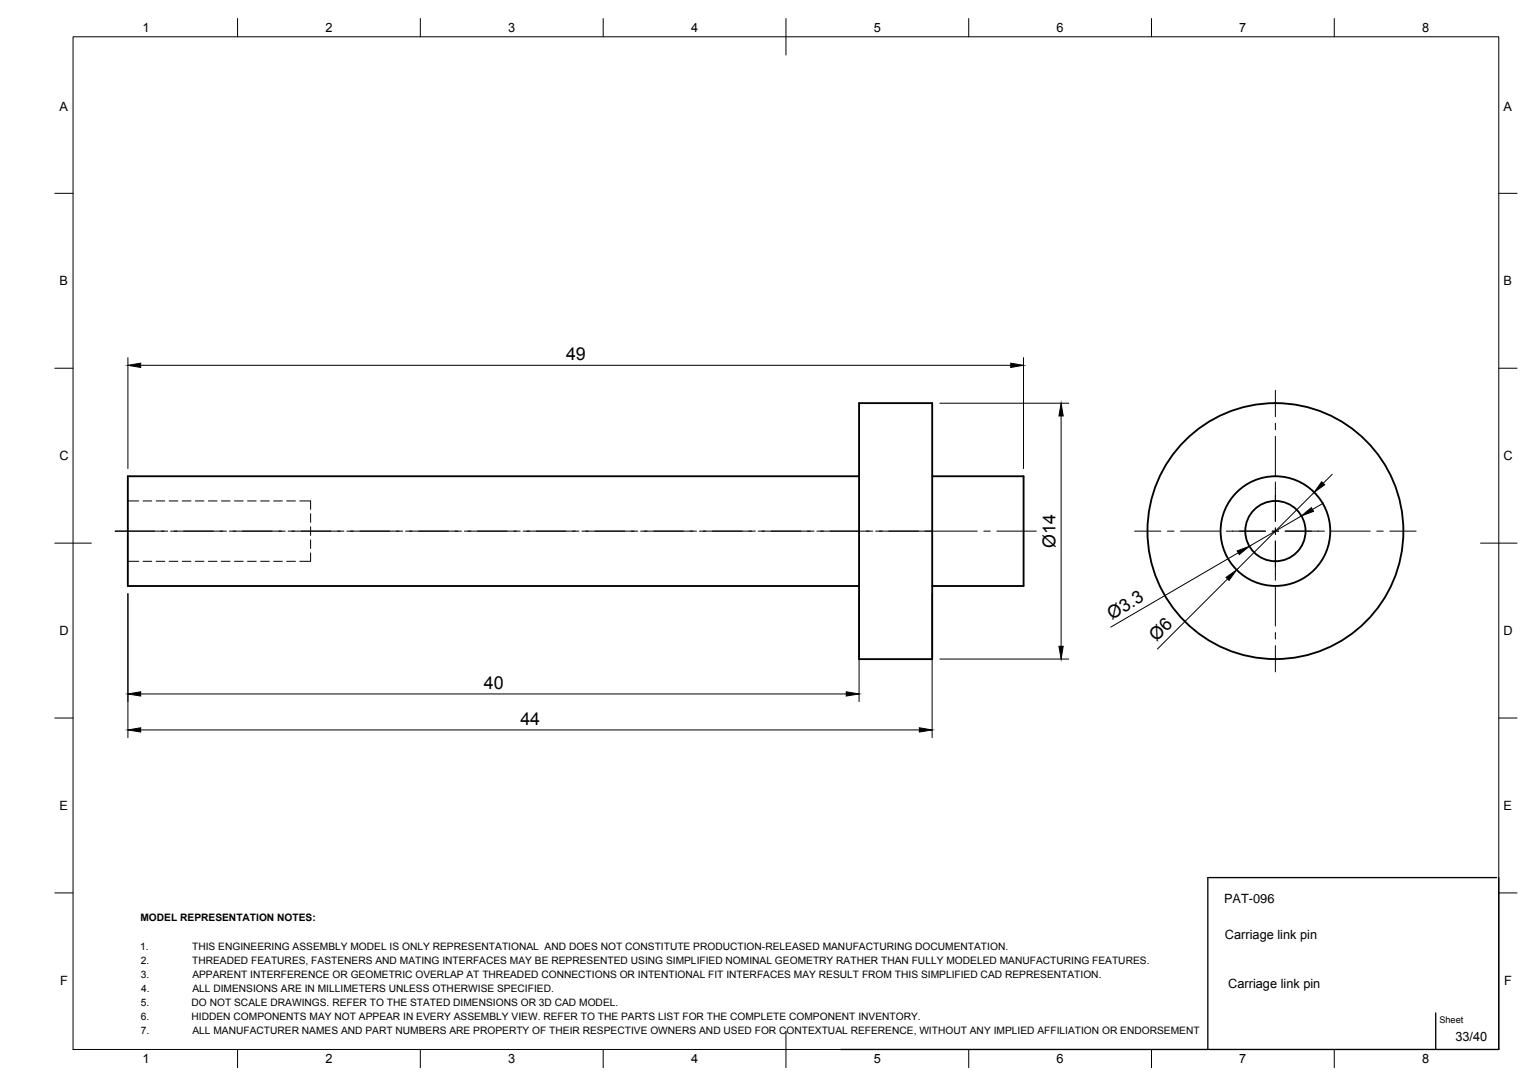
ISO-10303-21;
HEADER;
/* Generated by software containing ST-Developer
 * from STEP Tools, Inc. (www.steptools.com) 
 */

FILE_DESCRIPTION(
/* description */ ('PAT-096'),
/* implementation_level */ '2;1');

FILE_NAME(
/* name */ 'Carriage link pin.step',
/* time_stamp */ '2026-10-29T17:03:14-07:00',
/* author */ (''),
/* organization */ (''),
/* preprocessor_version */ 'ST-DEVELOPER v20.2',
/* originating_system */ 'Autodesk Translation Framework v15.17.0.0',
/* authorisation */ '');

FILE_SCHEMA (('AUTOMOTIVE_DESIGN { 1 0 10303 214 3 1 1 }'));
ENDSEC;

DATA;
#10=MECHANICAL_DESIGN_GEOMETRIC_PRESENTATION_REPRESENTATION('',(#428),#10650);
#358=SHAPE_REPRESENTATION_RELATIONSHIP('SRR','None',#10822,#389);
#389=ADVANCED_BREP_SHAPE_REPRESENTATION('',(#465),#10640);
#428=STYLED_ITEM('',(#11064),#465);
#465=MANIFOLD_SOLID_BREP('Body1',#5563);
#570=FACE_BOUND('',#1476,.T.);
#571=FACE_BOUND('',#1478,.T.);
#572=FACE_BOUND('',#1483,.T.);
#738=PLANE('',#6453);
#739=PLANE('',#6454);
#740=PLANE('',#6457);
#741=PLANE('',#6465);
#742=PLANE('',#6466);
#1040=FACE_OUTER_BOUND('',#1473,.T.);
#1041=FACE_OUTER_BOUND('',#1474,.T.);
#1042=FACE_OUTER_BOUND('',#1475,.T.);
#1043=FACE_OUTER_BOUND('',#1477,.T.);
#1044=FACE_OUTER_BOUND('',#1479,.T.);
#1045=FACE_OUTER_BOUND('',#1480,.T.);
#1046=FACE_OUTER_BOUND('',#1481,.T.);
#1047=FACE_OUTER_BOUND('',#1482,.T.);
#1048=FACE_OUTER_BOUND('',#1484,.T.);
#1473=EDGE_LOOP('',(#4743,#4744,#4745,#4746));
#1474=EDGE_LOOP('',(#4747));
#1475=EDGE_LOOP('',(#4748));
#1476=EDGE_LOOP('',(#4749));
#1477=EDGE_LOOP('',(#4750));
#1478=EDGE_LOOP('',(#4751));
#1479=EDGE_LOOP('',(#4752,#4753,#4754,#4755));
#1480=EDGE_LOOP('',(#4756,#4757,#4758,#4759));
#1481=EDGE_LOOP('',(#4760,#4761,#4762,#4763));
#1482=EDGE_LOOP('',(#4764));
#1483=EDGE_LOOP('',(#4765));
#1484=EDGE_LOOP('',(#4766));
#1836=LINE('',#10153,#2165);
#1837=LINE('',#10167,#2166);
#1838=LINE('',#10170,#2167);
#1839=LINE('',#10175,#2168);
#2165=VECTOR('',#7980,0.165);
#2166=VECTOR('',#7999,0.699999999999999);
#2167=VECTOR('',#8002,0.3);
#2168=VECTOR('',#8009,0.3);
#2507=CIRCLE('',#6451,0.165);
#2508=CIRCLE('',#6452,0.165);
#2509=CIRCLE('',#6455,0.699999999999999);
#2510=CIRCLE('',#6456,0.3);
#2511=CIRCLE('',#6458,0.699999999999999);
#2512=CIRCLE('',#6459,0.3);
#2513=CIRCLE('',#6462,0.3);
#2514=CIRCLE('',#6464,0.3);
#2927=VERTEX_POINT('',#10150);
#2928=VERTEX_POINT('',#10152);
#2929=VERTEX_POINT('',#10157);
#2930=VERTEX_POINT('',#10159);
#2931=VERTEX_POINT('',#10162);
#2932=VERTEX_POINT('',#10164);
#2933=VERTEX_POINT('',#10169);
#2934=VERTEX_POINT('',#10173);
#3550=EDGE_CURVE('',#2927,#2927,#2507,.T.);
#3551=EDGE_CURVE('',#2927,#2928,#1836,.T.);
#3552=EDGE_CURVE('',#2928,#2928,#2508,.T.);
#3553=EDGE_CURVE('',#2929,#2929,#2509,.T.);
#3554=EDGE_CURVE('',#2930,#2930,#2510,.T.);
#3555=EDGE_CURVE('',#2931,#2931,#2511,.T.);
#3556=EDGE_CURVE('',#2932,#2932,#2512,.T.);
#3557=EDGE_CURVE('',#2929,#2931,#1837,.T.);
#3558=EDGE_CURVE('',#2932,#2933,#1838,.T.);
#3559=EDGE_CURVE('',#2933,#2933,#2513,.T.);
#3560=EDGE_CURVE('',#2934,#2934,#2514,.T.);
#3561=EDGE_CURVE('',#2934,#2930,#1839,.T.);
#4743=ORIENTED_EDGE('',*,*,#3550,.F.);
#4744=ORIENTED_EDGE('',*,*,#3551,.T.);
#4745=ORIENTED_EDGE('',*,*,#3552,.F.);
#4746=ORIENTED_EDGE('',*,*,#3551,.F.);
#4747=ORIENTED_EDGE('',*,*,#3550,.T.);
#4748=ORIENTED_EDGE('',*,*,#3553,.T.);
#4749=ORIENTED_EDGE('',*,*,#3554,.F.);
#4750=ORIENTED_EDGE('',*,*,#3555,.F.);
#4751=ORIENTED_EDGE('',*,*,#3556,.F.);
#4752=ORIENTED_EDGE('',*,*,#3553,.F.);
#4753=ORIENTED_EDGE('',*,*,#3557,.T.);
#4754=ORIENTED_EDGE('',*,*,#3555,.T.);
#4755=ORIENTED_EDGE('',*,*,#3557,.F.);
#4756=ORIENTED_EDGE('',*,*,#3556,.T.);
#4757=ORIENTED_EDGE('',*,*,#3558,.T.);
#4758=ORIENTED_EDGE('',*,*,#3559,.T.);
#4759=ORIENTED_EDGE('',*,*,#3558,.F.);
#4760=ORIENTED_EDGE('',*,*,#3560,.F.);
#4761=ORIENTED_EDGE('',*,*,#3561,.T.);
#4762=ORIENTED_EDGE('',*,*,#3554,.T.);
#4763=ORIENTED_EDGE('',*,*,#3561,.F.);
#4764=ORIENTED_EDGE('',*,*,#3560,.T.);
#4765=ORIENTED_EDGE('',*,*,#3552,.T.);
#4766=ORIENTED_EDGE('',*,*,#3559,.F.);
#5164=CYLINDRICAL_SURFACE('',#6450,0.165);
#5165=CYLINDRICAL_SURFACE('',#6460,0.699999999999999);
#5166=CYLINDRICAL_SURFACE('',#6461,0.3);
#5167=CYLINDRICAL_SURFACE('',#6463,0.3);
#5445=ADVANCED_FACE('',(#1040),#5164,.F.);
#5446=ADVANCED_FACE('',(#1041),#738,.T.);
#5447=ADVANCED_FACE('',(#1042,#570),#739,.T.);
#5448=ADVANCED_FACE('',(#1043,#571),#740,.F.);
#5449=ADVANCED_FACE('',(#1044),#5165,.T.);
#5450=ADVANCED_FACE('',(#1045),#5166,.T.);
#5451=ADVANCED_FACE('',(#1046),#5167,.T.);
#5452=ADVANCED_FACE('',(#1047,#572),#741,.T.);
#5453=ADVANCED_FACE('',(#1048),#742,.F.);
#5563=CLOSED_SHELL('',(#5445,#5446,#5447,#5448,#5449,#5450,#5451,#5452,
#5453));
#6449=AXIS2_PLACEMENT_3D('',#10148,#7974,#7975);
#6450=AXIS2_PLACEMENT_3D('',#10149,#7976,#7977);
#6451=AXIS2_PLACEMENT_3D('',#10151,#7978,#7979);
#6452=AXIS2_PLACEMENT_3D('',#10154,#7981,#7982);
#6453=AXIS2_PLACEMENT_3D('',#10155,#7983,#7984);
#6454=AXIS2_PLACEMENT_3D('',#10156,#7985,#7986);
#6455=AXIS2_PLACEMENT_3D('',#10158,#7987,#7988);
#6456=AXIS2_PLACEMENT_3D('',#10160,#7989,#7990);
#6457=AXIS2_PLACEMENT_3D('',#10161,#7991,#7992);
#6458=AXIS2_PLACEMENT_3D('',#10163,#7993,#7994);
#6459=AXIS2_PLACEMENT_3D('',#10165,#7995,#7996);
#6460=AXIS2_PLACEMENT_3D('',#10166,#7997,#7998);
#6461=AXIS2_PLACEMENT_3D('',#10168,#8000,#8001);
#6462=AXIS2_PLACEMENT_3D('',#10171,#8003,#8004);
#6463=AXIS2_PLACEMENT_3D('',#10172,#8005,#8006);
#6464=AXIS2_PLACEMENT_3D('',#10174,#8007,#8008);
#6465=AXIS2_PLACEMENT_3D('',#10176,#8010,#8011);
#6466=AXIS2_PLACEMENT_3D('',#10177,#8012,#8013);
#7974=DIRECTION('axis',(0.,0.,1.));
#7975=DIRECTION('refdir',(1.,0.,0.));
#7976=DIRECTION('center_axis',(0.,0.,1.));
#7977=DIRECTION('ref_axis',(1.,0.,0.));
#7978=DIRECTION('center_axis',(0.,0.,1.));
#7979=DIRECTION('ref_axis',(1.,0.,0.));
#7980=DIRECTION('',(0.,0.,1.));
#7981=DIRECTION('center_axis',(0.,0.,-1.));
#7982=DIRECTION('ref_axis',(1.,0.,0.));
#7983=DIRECTION('center_axis',(0.,0.,1.));
#7984=DIRECTION('ref_axis',(1.,0.,0.));
#7985=DIRECTION('center_axis',(0.,0.,1.));
#7986=DIRECTION('ref_axis',(1.,0.,0.));
#7987=DIRECTION('center_axis',(0.,0.,1.));
#7988=DIRECTION('ref_axis',(1.,0.,0.));
#7989=DIRECTION('center_axis',(0.,0.,1.));
#7990=DIRECTION('ref_axis',(1.,0.,0.));
#7991=DIRECTION('center_axis',(0.,0.,1.));
#7992=DIRECTION('ref_axis',(1.,0.,0.));
#7993=DIRECTION('center_axis',(0.,0.,1.));
#7994=DIRECTION('ref_axis',(1.,0.,0.));
#7995=DIRECTION('center_axis',(0.,0.,-1.));
#7996=DIRECTION('ref_axis',(1.,0.,0.));
#7997=DIRECTION('center_axis',(0.,0.,1.));
#7998=DIRECTION('ref_axis',(1.,0.,0.));
#7999=DIRECTION('',(0.,0.,-1.));
#8000=DIRECTION('center_axis',(0.,0.,1.));
#8001=DIRECTION('ref_axis',(1.,0.,0.));
#8002=DIRECTION('',(0.,0.,-1.));
#8003=DIRECTION('center_axis',(0.,0.,1.));
#8004=DIRECTION('ref_axis',(1.,0.,0.));
#8005=DIRECTION('center_axis',(0.,0.,1.));
#8006=DIRECTION('ref_axis',(1.,0.,0.));
#8007=DIRECTION('center_axis',(0.,0.,1.));
#8008=DIRECTION('ref_axis',(1.,0.,0.));
#8009=DIRECTION('',(0.,0.,-1.));
#8010=DIRECTION('center_axis',(0.,0.,1.));
#8011=DIRECTION('ref_axis',(1.,0.,0.));
#8012=DIRECTION('center_axis',(0.,0.,1.));
#8013=DIRECTION('ref_axis',(1.,0.,0.));
#10148=CARTESIAN_POINT('',(0.,0.,0.));
#10149=CARTESIAN_POINT('Origin',(7.5,4.,9.1));
#10150=CARTESIAN_POINT('',(7.335,4.,9.1));
#10151=CARTESIAN_POINT('Origin',(7.5,4.,9.1));
#10152=CARTESIAN_POINT('',(7.335,4.,10.1));
#10153=CARTESIAN_POINT('',(7.335,4.,9.1));
#10154=CARTESIAN_POINT('Origin',(7.5,4.,10.1));
#10155=CARTESIAN_POINT('Origin',(7.5,4.,9.1));
#10156=CARTESIAN_POINT('Origin',(7.5,4.,6.1));
#10157=CARTESIAN_POINT('',(6.8,4.,6.1));
#10158=CARTESIAN_POINT('Origin',(7.5,4.,6.1));
#10159=CARTESIAN_POINT('',(7.2,4.,6.1));
#10160=CARTESIAN_POINT('Origin',(7.5,4.,6.1));
#10161=CARTESIAN_POINT('Origin',(7.5,4.,5.7));
#10162=CARTESIAN_POINT('',(6.8,4.,5.7));
#10163=CARTESIAN_POINT('Origin',(7.5,4.,5.7));
#10164=CARTESIAN_POINT('',(7.2,4.,5.7));
#10165=CARTESIAN_POINT('Origin',(7.5,4.,5.7));
#10166=CARTESIAN_POINT('Origin',(7.5,4.,5.7));
#10167=CARTESIAN_POINT('',(6.8,4.,5.7));
#10168=CARTESIAN_POINT('Origin',(7.5,4.,5.2));
#10169=CARTESIAN_POINT('',(7.2,4.,5.2));
#10170=CARTESIAN_POINT('',(7.2,4.,5.2));
#10171=CARTESIAN_POINT('Origin',(7.5,4.,5.2));
#10172=CARTESIAN_POINT('Origin',(7.5,4.,5.2));
#10173=CARTESIAN_POINT('',(7.2,4.,10.1));
#10174=CARTESIAN_POINT('Origin',(7.5,4.,10.1));
#10175=CARTESIAN_POINT('',(7.2,4.,5.2));
#10176=CARTESIAN_POINT('Origin',(7.5,4.,10.1));
#10177=CARTESIAN_POINT('Origin',(7.5,4.,5.2));
#10601=UNCERTAINTY_MEASURE_WITH_UNIT(LENGTH_MEASURE(0.001),#10651,
'DISTANCE_ACCURACY_VALUE',
'Maximum model space distance between geometric entities at asserted c
onnectivities');
#10611=UNCERTAINTY_MEASURE_WITH_UNIT(LENGTH_MEASURE(0.001),#10651,
'DISTANCE_ACCURACY_VALUE',
'Maximum model space distance between geometric entities at asserted c
onnectivities');
#10640=(
GEOMETRIC_REPRESENTATION_CONTEXT(3)
GLOBAL_UNCERTAINTY_ASSIGNED_CONTEXT((#10601))
GLOBAL_UNIT_ASSIGNED_CONTEXT((#10651,#10653,#10654))
REPRESENTATION_CONTEXT('','3D')
);
#10650=(
GEOMETRIC_REPRESENTATION_CONTEXT(3)
GLOBAL_UNCERTAINTY_ASSIGNED_CONTEXT((#10611))
GLOBAL_UNIT_ASSIGNED_CONTEXT((#10651,#10653,#10654))
REPRESENTATION_CONTEXT('','3D')
);
#10651=(
LENGTH_UNIT()
NAMED_UNIT(*)
SI_UNIT(.CENTI.,.METRE.)
);
#10653=(
NAMED_UNIT(*)
PLANE_ANGLE_UNIT()
SI_UNIT($,.RADIAN.)
);
#10654=(
NAMED_UNIT(*)
SI_UNIT($,.STERADIAN.)
SOLID_ANGLE_UNIT()
);
#10683=SHAPE_DEFINITION_REPRESENTATION(#10729,#10822);
#10729=PRODUCT_DEFINITION_SHAPE('',$,#10861);
#10822=SHAPE_REPRESENTATION('',(#6449),#10640);
#10832=PRODUCT_DEFINITION_CONTEXT('part definition',#10948,'design');
#10861=PRODUCT_DEFINITION('Carriage link pin','Carriage link pin',#10899,
#10832);
#10899=PRODUCT_DEFINITION_FORMATION('',$,#10978);
#10948=APPLICATION_CONTEXT(
'Core Data for Automotive Mechanical Design Process');
#10949=PRODUCT_CONTEXT('part definition',#10948,'mechanical');
#10978=PRODUCT('Carriage link pin','Carriage link pin',
'Carriage link pin',(#10949));
#11058=COLOUR_RGB('Grey',0.48,0.52,0.57);
#11059=FILL_AREA_STYLE_COLOUR('',#11058);
#11060=FILL_AREA_STYLE('',(#11059));
#11061=SURFACE_STYLE_FILL_AREA(#11060);
#11062=SURFACE_SIDE_STYLE('',(#11061));
#11063=SURFACE_STYLE_USAGE(.BOTH.,#11062);
#11064=PRESENTATION_STYLE_ASSIGNMENT((#11063));
ENDSEC;
END-ISO-10303-21;
